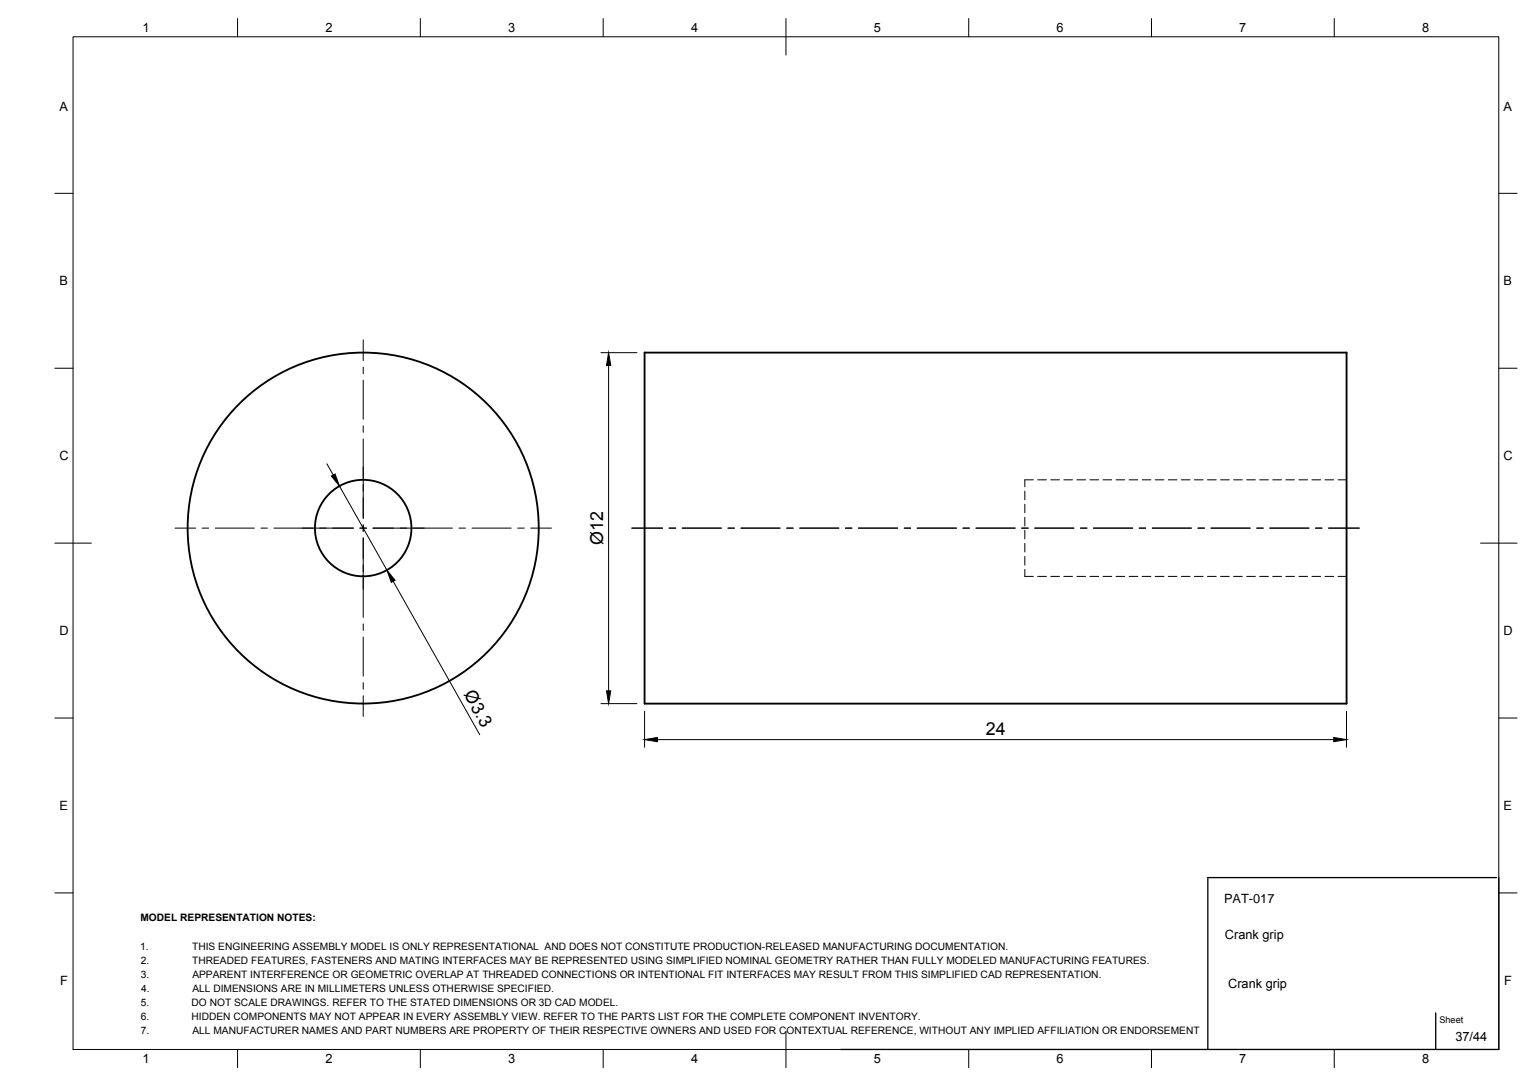
ISO-10303-21;
HEADER;
/* Generated by software containing ST-Developer
 * from STEP Tools, Inc. (www.steptools.com) 
 */

FILE_DESCRIPTION(
/* description */ ('Cam-and-follower valve demonstrator'),
/* implementation_level */ '2;1');

FILE_NAME(
/* name */ 'Crank grip.step',
/* time_stamp */ '2026-10-28T03:25:17-07:00',
/* author */ (''),
/* organization */ (''),
/* preprocessor_version */ 'ST-DEVELOPER v20.2',
/* originating_system */ 'Autodesk Translation Framework v15.17.0.0',
/* authorisation */ '');

FILE_SCHEMA (('AUTOMOTIVE_DESIGN { 1 0 10303 214 3 1 1 }'));
ENDSEC;

DATA;
#10=MECHANICAL_DESIGN_GEOMETRIC_PRESENTATION_REPRESENTATION('',(#447),#12896);
#368=SHAPE_REPRESENTATION_RELATIONSHIP('SRR','None',#13087,#404);
#404=ADVANCED_BREP_SHAPE_REPRESENTATION('',(#488),#12887);
#447=STYLED_ITEM('',(#13337),#488);
#488=MANIFOLD_SOLID_BREP('Body1',#6216);
#647=FACE_BOUND('',#1930,.T.);
#941=CIRCLE('',#7255,0.165);
#942=CIRCLE('',#7256,0.165);
#943=CIRCLE('',#7259,0.6);
#944=CIRCLE('',#7260,0.6);
#1081=CYLINDRICAL_SURFACE('',#7254,0.165);
#1082=CYLINDRICAL_SURFACE('',#7258,0.6);
#1405=FACE_OUTER_BOUND('',#1925,.T.);
#1406=FACE_OUTER_BOUND('',#1926,.T.);
#1407=FACE_OUTER_BOUND('',#1927,.T.);
#1408=FACE_OUTER_BOUND('',#1928,.T.);
#1409=FACE_OUTER_BOUND('',#1929,.T.);
#1925=EDGE_LOOP('',(#5389,#5390,#5391,#5392));
#1926=EDGE_LOOP('',(#5393));
#1927=EDGE_LOOP('',(#5394,#5395,#5396,#5397));
#1928=EDGE_LOOP('',(#5398));
#1929=EDGE_LOOP('',(#5399));
#1930=EDGE_LOOP('',(#5400));
#2345=LINE('',#12515,#2767);
#2346=LINE('',#12522,#2768);
#2767=VECTOR('',#9032,0.165);
#2768=VECTOR('',#9041,0.6);
#3276=VERTEX_POINT('',#12512);
#3277=VERTEX_POINT('',#12514);
#3278=VERTEX_POINT('',#12519);
#3279=VERTEX_POINT('',#12521);
#3991=EDGE_CURVE('',#3276,#3276,#941,.T.);
#3992=EDGE_CURVE('',#3276,#3277,#2345,.T.);
#3993=EDGE_CURVE('',#3277,#3277,#942,.T.);
#3994=EDGE_CURVE('',#3278,#3278,#943,.T.);
#3995=EDGE_CURVE('',#3278,#3279,#2346,.T.);
#3996=EDGE_CURVE('',#3279,#3279,#944,.T.);
#5389=ORIENTED_EDGE('',*,*,#3991,.F.);
#5390=ORIENTED_EDGE('',*,*,#3992,.T.);
#5391=ORIENTED_EDGE('',*,*,#3993,.T.);
#5392=ORIENTED_EDGE('',*,*,#3992,.F.);
#5393=ORIENTED_EDGE('',*,*,#3993,.F.);
#5394=ORIENTED_EDGE('',*,*,#3994,.F.);
#5395=ORIENTED_EDGE('',*,*,#3995,.T.);
#5396=ORIENTED_EDGE('',*,*,#3996,.T.);
#5397=ORIENTED_EDGE('',*,*,#3995,.F.);
#5398=ORIENTED_EDGE('',*,*,#3994,.T.);
#5399=ORIENTED_EDGE('',*,*,#3996,.F.);
#5400=ORIENTED_EDGE('',*,*,#3991,.T.);
#5771=PLANE('',#7257);
#5772=PLANE('',#7261);
#5773=PLANE('',#7262);
#6121=ADVANCED_FACE('',(#1405),#1081,.F.);
#6122=ADVANCED_FACE('',(#1406),#5771,.F.);
#6123=ADVANCED_FACE('',(#1407),#1082,.T.);
#6124=ADVANCED_FACE('',(#1408),#5772,.T.);
#6125=ADVANCED_FACE('',(#1409,#647),#5773,.F.);
#6216=CLOSED_SHELL('',(#6121,#6122,#6123,#6124,#6125));
#7253=AXIS2_PLACEMENT_3D('',#12510,#9026,#9027);
#7254=AXIS2_PLACEMENT_3D('',#12511,#9028,#9029);
#7255=AXIS2_PLACEMENT_3D('',#12513,#9030,#9031);
#7256=AXIS2_PLACEMENT_3D('',#12516,#9033,#9034);
#7257=AXIS2_PLACEMENT_3D('',#12517,#9035,#9036);
#7258=AXIS2_PLACEMENT_3D('',#12518,#9037,#9038);
#7259=AXIS2_PLACEMENT_3D('',#12520,#9039,#9040);
#7260=AXIS2_PLACEMENT_3D('',#12523,#9042,#9043);
#7261=AXIS2_PLACEMENT_3D('',#12524,#9044,#9045);
#7262=AXIS2_PLACEMENT_3D('',#12525,#9046,#9047);
#9026=DIRECTION('axis',(0.,0.,1.));
#9027=DIRECTION('refdir',(1.,0.,0.));
#9028=DIRECTION('center_axis',(0.,1.,0.));
#9029=DIRECTION('ref_axis',(1.,0.,0.));
#9030=DIRECTION('center_axis',(0.,1.,0.));
#9031=DIRECTION('ref_axis',(1.,0.,0.));
#9032=DIRECTION('',(0.,1.,0.));
#9033=DIRECTION('center_axis',(0.,1.,0.));
#9034=DIRECTION('ref_axis',(1.,0.,0.));
#9035=DIRECTION('center_axis',(0.,1.,0.));
#9036=DIRECTION('ref_axis',(1.,0.,0.));
#9037=DIRECTION('center_axis',(0.,1.,0.));
#9038=DIRECTION('ref_axis',(1.,0.,0.));
#9039=DIRECTION('center_axis',(0.,1.,0.));
#9040=DIRECTION('ref_axis',(1.,0.,0.));
#9041=DIRECTION('',(0.,-1.,0.));
#9042=DIRECTION('center_axis',(0.,1.,0.));
#9043=DIRECTION('ref_axis',(1.,0.,0.));
#9044=DIRECTION('center_axis',(0.,1.,0.));
#9045=DIRECTION('ref_axis',(1.,0.,0.));
#9046=DIRECTION('center_axis',(0.,1.,0.));
#9047=DIRECTION('ref_axis',(1.,0.,0.));
#12510=CARTESIAN_POINT('',(0.,0.,0.));
#12511=CARTESIAN_POINT('Origin',(2.5,5.7,4.));
#12512=CARTESIAN_POINT('',(2.335,5.8,4.));
#12513=CARTESIAN_POINT('Origin',(2.5,5.8,4.));
#12514=CARTESIAN_POINT('',(2.335,6.9,4.));
#12515=CARTESIAN_POINT('',(2.335,5.7,4.));
#12516=CARTESIAN_POINT('Origin',(2.5,6.9,4.));
#12517=CARTESIAN_POINT('Origin',(2.5,6.9,4.));
#12518=CARTESIAN_POINT('Origin',(2.5,5.8,4.));
#12519=CARTESIAN_POINT('',(1.9,8.2,4.));
#12520=CARTESIAN_POINT('Origin',(2.5,8.2,4.));
#12521=CARTESIAN_POINT('',(1.9,5.8,4.));
#12522=CARTESIAN_POINT('',(1.9,5.8,4.));
#12523=CARTESIAN_POINT('Origin',(2.5,5.8,4.));
#12524=CARTESIAN_POINT('Origin',(2.5,8.2,4.));
#12525=CARTESIAN_POINT('Origin',(2.5,5.8,4.));
#12844=UNCERTAINTY_MEASURE_WITH_UNIT(LENGTH_MEASURE(0.001),#12897,
'DISTANCE_ACCURACY_VALUE',
'Maximum model space distance between geometric entities at asserted c
onnectivities');
#12853=UNCERTAINTY_MEASURE_WITH_UNIT(LENGTH_MEASURE(0.001),#12897,
'DISTANCE_ACCURACY_VALUE',
'Maximum model space distance between geometric entities at asserted c
onnectivities');
#12887=(
GEOMETRIC_REPRESENTATION_CONTEXT(3)
GLOBAL_UNCERTAINTY_ASSIGNED_CONTEXT((#12844))
GLOBAL_UNIT_ASSIGNED_CONTEXT((#12897,#12899,#12900))
REPRESENTATION_CONTEXT('','3D')
);
#12896=(
GEOMETRIC_REPRESENTATION_CONTEXT(3)
GLOBAL_UNCERTAINTY_ASSIGNED_CONTEXT((#12853))
GLOBAL_UNIT_ASSIGNED_CONTEXT((#12897,#12899,#12900))
REPRESENTATION_CONTEXT('','3D')
);
#12897=(
LENGTH_UNIT()
NAMED_UNIT(*)
SI_UNIT(.CENTI.,.METRE.)
);
#12899=(
NAMED_UNIT(*)
PLANE_ANGLE_UNIT()
SI_UNIT($,.RADIAN.)
);
#12900=(
NAMED_UNIT(*)
SI_UNIT($,.STERADIAN.)
SOLID_ANGLE_UNIT()
);
#12934=SHAPE_DEFINITION_REPRESENTATION(#12983,#13087);
#12983=PRODUCT_DEFINITION_SHAPE('',$,#13130);
#13087=SHAPE_REPRESENTATION('',(#7253),#12887);
#13096=PRODUCT_DEFINITION_CONTEXT('part definition',#13224,'design');
#13130=PRODUCT_DEFINITION('Crank grip','Crank grip',#13172,#13096);
#13172=PRODUCT_DEFINITION_FORMATION('',$,#13259);
#13224=APPLICATION_CONTEXT(
'Core Data for Automotive Mechanical Design Process');
#13225=PRODUCT_CONTEXT('part definition',#13224,'mechanical');
#13259=PRODUCT('Crank grip','Crank grip','Crank grip',(#13225));
#13331=COLOUR_RGB('Black',0.12,0.14,0.17);
#13332=FILL_AREA_STYLE_COLOUR('',#13331);
#13333=FILL_AREA_STYLE('',(#13332));
#13334=SURFACE_STYLE_FILL_AREA(#13333);
#13335=SURFACE_SIDE_STYLE('',(#13334));
#13336=SURFACE_STYLE_USAGE(.BOTH.,#13335);
#13337=PRESENTATION_STYLE_ASSIGNMENT((#13336));
ENDSEC;
END-ISO-10303-21;
